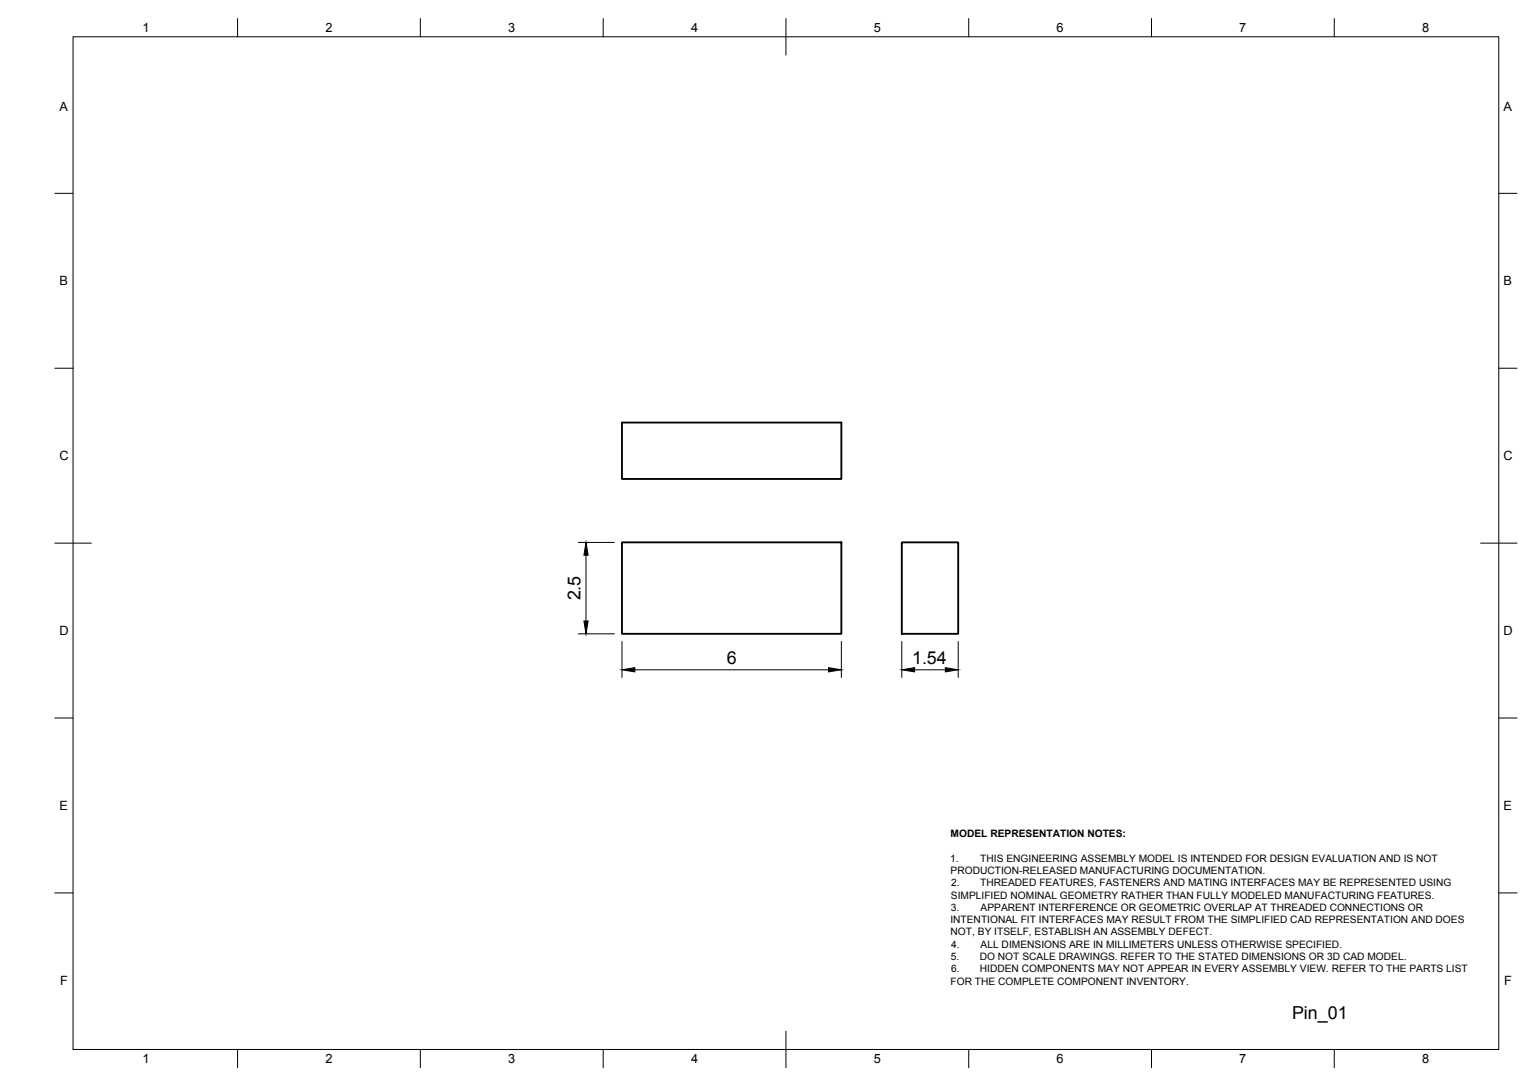
ISO-10303-21;
HEADER;
/* Generated by software containing ST-Developer
 * from STEP Tools, Inc. (www.steptools.com) 
 */

FILE_DESCRIPTION(
/* description */ (''),
/* implementation_level */ '2;1');

FILE_NAME(
/* name */ 'Pin_01.step',
/* time_stamp */ '2026-10-05T22:24:12-07:00',
/* author */ (''),
/* organization */ (''),
/* preprocessor_version */ 'ST-DEVELOPER v20.2',
/* originating_system */ 'Autodesk Translation Framework v15.15.0.0',
/* authorisation */ '');

FILE_SCHEMA (('AUTOMOTIVE_DESIGN { 1 0 10303 214 3 1 1 }'));
ENDSEC;

DATA;
#10=MECHANICAL_DESIGN_GEOMETRIC_PRESENTATION_REPRESENTATION('',(#59),#2116);
#45=SHAPE_REPRESENTATION_RELATIONSHIP('SRR','None',#2151,#52);
#52=ADVANCED_BREP_SHAPE_REPRESENTATION('',(#66),#2115);
#59=STYLED_ITEM('',(#2192),#66);
#66=MANIFOLD_SOLID_BREP('Body1',#1153);
#125=PLANE('',#1341);
#126=PLANE('',#1342);
#127=PLANE('',#1343);
#128=PLANE('',#1344);
#129=PLANE('',#1345);
#130=PLANE('',#1346);
#192=FACE_OUTER_BOUND('',#267,.T.);
#193=FACE_OUTER_BOUND('',#268,.T.);
#194=FACE_OUTER_BOUND('',#269,.T.);
#195=FACE_OUTER_BOUND('',#270,.T.);
#196=FACE_OUTER_BOUND('',#271,.T.);
#197=FACE_OUTER_BOUND('',#272,.T.);
#267=EDGE_LOOP('',(#1045,#1046,#1047,#1048));
#268=EDGE_LOOP('',(#1049,#1050,#1051,#1052));
#269=EDGE_LOOP('',(#1053,#1054,#1055,#1056));
#270=EDGE_LOOP('',(#1057,#1058,#1059,#1060));
#271=EDGE_LOOP('',(#1061,#1062,#1063,#1064));
#272=EDGE_LOOP('',(#1065,#1066,#1067,#1068));
#369=LINE('',#2069,#474);
#370=LINE('',#2071,#475);
#371=LINE('',#2073,#476);
#372=LINE('',#2074,#477);
#373=LINE('',#2077,#478);
#374=LINE('',#2079,#479);
#375=LINE('',#2080,#480);
#376=LINE('',#2083,#481);
#377=LINE('',#2085,#482);
#378=LINE('',#2086,#483);
#379=LINE('',#2088,#484);
#380=LINE('',#2089,#485);
#474=VECTOR('',#1667,10.);
#475=VECTOR('',#1668,10.);
#476=VECTOR('',#1669,10.);
#477=VECTOR('',#1670,10.);
#478=VECTOR('',#1673,10.);
#479=VECTOR('',#1674,10.);
#480=VECTOR('',#1675,10.);
#481=VECTOR('',#1678,10.);
#482=VECTOR('',#1679,10.);
#483=VECTOR('',#1680,10.);
#484=VECTOR('',#1683,10.);
#485=VECTOR('',#1684,10.);
#617=VERTEX_POINT('',#2067);
#618=VERTEX_POINT('',#2068);
#619=VERTEX_POINT('',#2070);
#620=VERTEX_POINT('',#2072);
#621=VERTEX_POINT('',#2076);
#622=VERTEX_POINT('',#2078);
#623=VERTEX_POINT('',#2082);
#624=VERTEX_POINT('',#2084);
#761=EDGE_CURVE('',#617,#618,#369,.T.);
#762=EDGE_CURVE('',#617,#619,#370,.T.);
#763=EDGE_CURVE('',#620,#619,#371,.T.);
#764=EDGE_CURVE('',#618,#620,#372,.T.);
#765=EDGE_CURVE('',#618,#621,#373,.T.);
#766=EDGE_CURVE('',#622,#620,#374,.T.);
#767=EDGE_CURVE('',#621,#622,#375,.T.);
#768=EDGE_CURVE('',#623,#621,#376,.T.);
#769=EDGE_CURVE('',#624,#622,#377,.T.);
#770=EDGE_CURVE('',#623,#624,#378,.T.);
#771=EDGE_CURVE('',#617,#623,#379,.T.);
#772=EDGE_CURVE('',#619,#624,#380,.T.);
#1045=ORIENTED_EDGE('',*,*,#761,.F.);
#1046=ORIENTED_EDGE('',*,*,#762,.T.);
#1047=ORIENTED_EDGE('',*,*,#763,.F.);
#1048=ORIENTED_EDGE('',*,*,#764,.F.);
#1049=ORIENTED_EDGE('',*,*,#765,.F.);
#1050=ORIENTED_EDGE('',*,*,#764,.T.);
#1051=ORIENTED_EDGE('',*,*,#766,.F.);
#1052=ORIENTED_EDGE('',*,*,#767,.F.);
#1053=ORIENTED_EDGE('',*,*,#768,.T.);
#1054=ORIENTED_EDGE('',*,*,#767,.T.);
#1055=ORIENTED_EDGE('',*,*,#769,.F.);
#1056=ORIENTED_EDGE('',*,*,#770,.F.);
#1057=ORIENTED_EDGE('',*,*,#771,.T.);
#1058=ORIENTED_EDGE('',*,*,#770,.T.);
#1059=ORIENTED_EDGE('',*,*,#772,.F.);
#1060=ORIENTED_EDGE('',*,*,#762,.F.);
#1061=ORIENTED_EDGE('',*,*,#772,.T.);
#1062=ORIENTED_EDGE('',*,*,#769,.T.);
#1063=ORIENTED_EDGE('',*,*,#766,.T.);
#1064=ORIENTED_EDGE('',*,*,#763,.T.);
#1065=ORIENTED_EDGE('',*,*,#771,.F.);
#1066=ORIENTED_EDGE('',*,*,#761,.T.);
#1067=ORIENTED_EDGE('',*,*,#765,.T.);
#1068=ORIENTED_EDGE('',*,*,#768,.F.);
#1141=ADVANCED_FACE('',(#192),#125,.T.);
#1142=ADVANCED_FACE('',(#193),#126,.T.);
#1143=ADVANCED_FACE('',(#194),#127,.T.);
#1144=ADVANCED_FACE('',(#195),#128,.T.);
#1145=ADVANCED_FACE('',(#196),#129,.T.);
#1146=ADVANCED_FACE('',(#197),#130,.F.);
#1153=CLOSED_SHELL('',(#1141,#1142,#1143,#1144,#1145,#1146));
#1340=AXIS2_PLACEMENT_3D('',#2065,#1663,#1664);
#1341=AXIS2_PLACEMENT_3D('',#2066,#1665,#1666);
#1342=AXIS2_PLACEMENT_3D('',#2075,#1671,#1672);
#1343=AXIS2_PLACEMENT_3D('',#2081,#1676,#1677);
#1344=AXIS2_PLACEMENT_3D('',#2087,#1681,#1682);
#1345=AXIS2_PLACEMENT_3D('',#2090,#1685,#1686);
#1346=AXIS2_PLACEMENT_3D('',#2091,#1687,#1688);
#1663=DIRECTION('axis',(0.,0.,1.));
#1664=DIRECTION('refdir',(1.,0.,0.));
#1665=DIRECTION('center_axis',(0.,0.,1.));
#1666=DIRECTION('ref_axis',(-1.,0.,0.));
#1667=DIRECTION('',(1.,0.,0.));
#1668=DIRECTION('',(0.,-1.,0.));
#1669=DIRECTION('',(-1.,0.,0.));
#1670=DIRECTION('',(0.,-1.,0.));
#1671=DIRECTION('center_axis',(1.,0.,0.));
#1672=DIRECTION('ref_axis',(0.,0.,1.));
#1673=DIRECTION('',(0.,0.,-1.));
#1674=DIRECTION('',(0.,0.,1.));
#1675=DIRECTION('',(0.,-1.,0.));
#1676=DIRECTION('center_axis',(0.,0.,-1.));
#1677=DIRECTION('ref_axis',(1.,0.,0.));
#1678=DIRECTION('',(1.,0.,0.));
#1679=DIRECTION('',(1.,0.,0.));
#1680=DIRECTION('',(0.,-1.,0.));
#1681=DIRECTION('center_axis',(-1.,0.,0.));
#1682=DIRECTION('ref_axis',(0.,0.,-1.));
#1683=DIRECTION('',(0.,0.,-1.));
#1684=DIRECTION('',(0.,0.,-1.));
#1685=DIRECTION('center_axis',(0.,-1.,0.));
#1686=DIRECTION('ref_axis',(0.,0.,-1.));
#1687=DIRECTION('center_axis',(0.,-1.,0.));
#1688=DIRECTION('ref_axis',(1.,0.,0.));
#2065=CARTESIAN_POINT('',(0.,0.,0.));
#2066=CARTESIAN_POINT('Origin',(1.25,-6.,4.84122918275927));
#2067=CARTESIAN_POINT('',(-1.25,-6.,4.84122918275927));
#2068=CARTESIAN_POINT('',(1.25,-6.,4.84122918275927));
#2069=CARTESIAN_POINT('',(-1.25,-6.,4.84122918275927));
#2070=CARTESIAN_POINT('',(-1.25,-12.,4.84122918275927));
#2071=CARTESIAN_POINT('',(-1.25,-6.,4.84122918275927));
#2072=CARTESIAN_POINT('',(1.25,-12.,4.84122918275927));
#2073=CARTESIAN_POINT('',(-1.25,-12.,4.84122918275927));
#2074=CARTESIAN_POINT('',(1.25,-6.,4.84122918275927));
#2075=CARTESIAN_POINT('Origin',(1.25,-6.,3.29967103839267));
#2076=CARTESIAN_POINT('',(1.25,-6.,3.29967103839267));
#2077=CARTESIAN_POINT('',(1.25,-6.,6.32461990770089));
#2078=CARTESIAN_POINT('',(1.25,-12.,3.29967103839267));
#2079=CARTESIAN_POINT('',(1.25,-12.,6.32461990770089));
#2080=CARTESIAN_POINT('',(1.25,-6.,3.29967103839267));
#2081=CARTESIAN_POINT('Origin',(-1.25,-6.,3.29967103839267));
#2082=CARTESIAN_POINT('',(-1.25,-6.,3.29967103839267));
#2083=CARTESIAN_POINT('',(-1.25,-6.,3.29967103839267));
#2084=CARTESIAN_POINT('',(-1.25,-12.,3.29967103839267));
#2085=CARTESIAN_POINT('',(-1.25,-12.,3.29967103839267));
#2086=CARTESIAN_POINT('',(-1.25,-6.,3.29967103839267));
#2087=CARTESIAN_POINT('Origin',(-1.25,-6.,4.84122918275927));
#2088=CARTESIAN_POINT('',(-1.25,-6.,3.79967103839267));
#2089=CARTESIAN_POINT('',(-1.25,-12.,3.79967103839267));
#2090=CARTESIAN_POINT('Origin',(0.,-12.,4.07045011057597));
#2091=CARTESIAN_POINT('Origin',(0.,-6.,4.07045011057597));
#2106=UNCERTAINTY_MEASURE_WITH_UNIT(LENGTH_MEASURE(0.01),#2117,
'DISTANCE_ACCURACY_VALUE',
'Maximum model space distance between geometric entities at asserted c
onnectivities');
#2107=UNCERTAINTY_MEASURE_WITH_UNIT(LENGTH_MEASURE(0.01),#2117,
'DISTANCE_ACCURACY_VALUE',
'Maximum model space distance between geometric entities at asserted c
onnectivities');
#2115=(
GEOMETRIC_REPRESENTATION_CONTEXT(3)
GLOBAL_UNCERTAINTY_ASSIGNED_CONTEXT((#2106))
GLOBAL_UNIT_ASSIGNED_CONTEXT((#2117,#2119,#2120))
REPRESENTATION_CONTEXT('','3D')
);
#2116=(
GEOMETRIC_REPRESENTATION_CONTEXT(3)
GLOBAL_UNCERTAINTY_ASSIGNED_CONTEXT((#2107))
GLOBAL_UNIT_ASSIGNED_CONTEXT((#2117,#2119,#2120))
REPRESENTATION_CONTEXT('','3D')
);
#2117=(
LENGTH_UNIT()
NAMED_UNIT(*)
SI_UNIT(.MILLI.,.METRE.)
);
#2119=(
NAMED_UNIT(*)
PLANE_ANGLE_UNIT()
SI_UNIT($,.RADIAN.)
);
#2120=(
NAMED_UNIT(*)
SI_UNIT($,.STERADIAN.)
SOLID_ANGLE_UNIT()
);
#2128=SHAPE_DEFINITION_REPRESENTATION(#2136,#2151);
#2136=PRODUCT_DEFINITION_SHAPE('',$,#2160);
#2151=SHAPE_REPRESENTATION('',(#1340),#2115);
#2152=PRODUCT_DEFINITION_CONTEXT('part definition',#2178,'design');
#2160=PRODUCT_DEFINITION('Pin_01','Pin_01',#2168,#2152);
#2168=PRODUCT_DEFINITION_FORMATION('',$,#2187);
#2178=APPLICATION_CONTEXT(
'Core Data for Automotive Mechanical Design Process');
#2179=PRODUCT_CONTEXT('part definition',#2178,'mechanical');
#2187=PRODUCT('Pin_01','Pin_01',$,(#2179));
#2192=PRESENTATION_STYLE_ASSIGNMENT((#2197));
#2197=SURFACE_STYLE_USAGE(.BOTH.,#2202);
#2202=SURFACE_SIDE_STYLE('',(#2207));
#2207=SURFACE_STYLE_FILL_AREA(#2212);
#2212=FILL_AREA_STYLE('Opaque(235,235,235)',(#2217));
#2217=FILL_AREA_STYLE_COLOUR('Opaque(235,235,235)',#2222);
#2222=COLOUR_RGB('Opaque(235,235,235)', 0.40784314, 0.44705882, 0.49803922);
ENDSEC;
END-ISO-10303-21;
